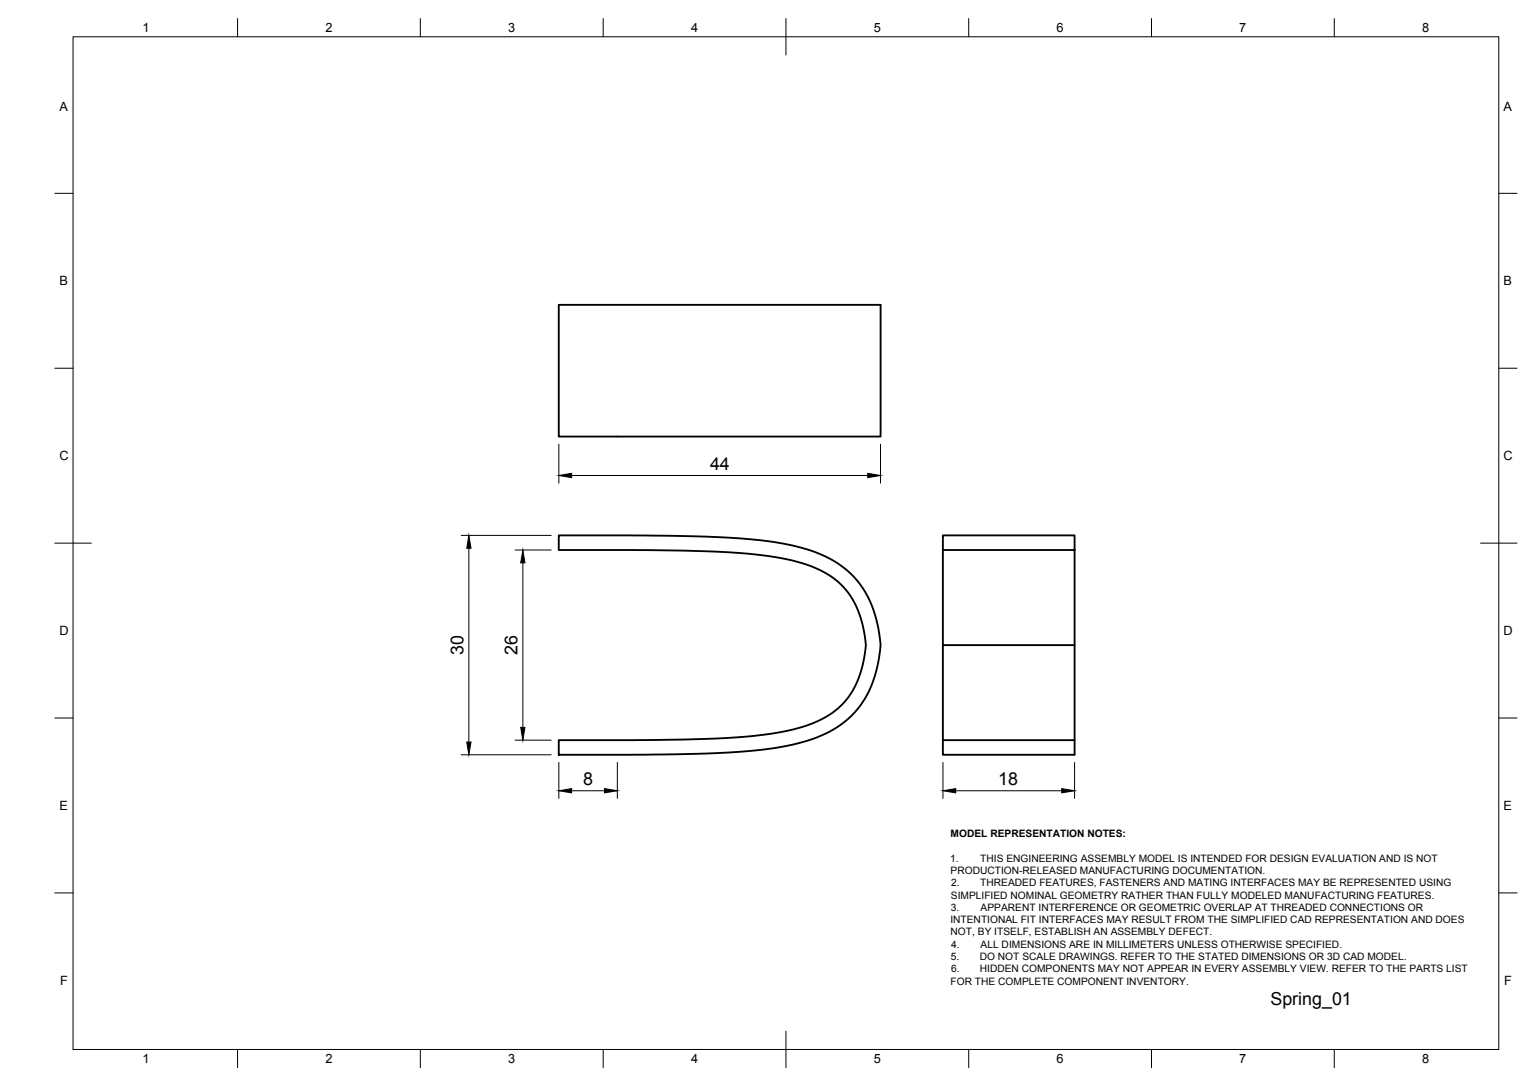
ISO-10303-21;
HEADER;
/* Generated by software containing ST-Developer
 * from STEP Tools, Inc. (www.steptools.com) 
 */

FILE_DESCRIPTION(
/* description */ (''),
/* implementation_level */ '2;1');

FILE_NAME(
/* name */ 'Spring_01.step',
/* time_stamp */ '2026-10-06T13:31:15-07:00',
/* author */ (''),
/* organization */ (''),
/* preprocessor_version */ 'ST-DEVELOPER v20.2',
/* originating_system */ 'Autodesk Translation Framework v15.15.0.0',
/* authorisation */ '');

FILE_SCHEMA (('AUTOMOTIVE_DESIGN { 1 0 10303 214 3 1 1 }'));
ENDSEC;

DATA;
#10=MECHANICAL_DESIGN_GEOMETRIC_PRESENTATION_REPRESENTATION('',(#85),#3154);
#55=B_SPLINE_SURFACE_WITH_KNOTS('',5,1,((#2342,#2343),(#2344,#2345),(#2346,
#2347),(#2348,#2349),(#2350,#2351),(#2352,#2353),(#2354,#2355),(#2356,#2357),
(#2358,#2359),(#2360,#2361),(#2362,#2363),(#2364,#2365),(#2366,#2367),(#2368,
#2369),(#2370,#2371),(#2372,#2373),(#2374,#2375),(#2376,#2377),(#2378,#2379),
(#2380,#2381)),.UNSPECIFIED.,.F.,.F.,.F.,(6,1,1,1,1,1,1,1,1,1,1,1,1,1,1,
6),(2,2),(-1.,-0.933333333333333,-0.866666666666667,-0.8,-0.733333333333333,
-0.666666666666667,-0.6,-0.533333333333333,-0.466666666666667,-0.4,-0.333333333333333,
-0.266666666666667,-0.2,-0.133333333333333,-0.0666666666666667,0.),(0.,
2.16),.UNSPECIFIED.);
#56=B_SPLINE_SURFACE_WITH_KNOTS('',5,1,((#2406,#2407),(#2408,#2409),(#2410,
#2411),(#2412,#2413),(#2414,#2415),(#2416,#2417),(#2418,#2419),(#2420,#2421),
(#2422,#2423),(#2424,#2425),(#2426,#2427),(#2428,#2429),(#2430,#2431),(#2432,
#2433),(#2434,#2435),(#2436,#2437),(#2438,#2439),(#2440,#2441),(#2442,#2443),
(#2444,#2445)),.UNSPECIFIED.,.F.,.F.,.F.,(6,1,1,1,1,1,1,1,1,1,1,1,1,1,1,
6),(2,2),(0.,0.0666666666666667,0.133333333333333,0.2,0.266666666666667,
0.333333333333333,0.4,0.466666666666667,0.533333333333333,0.6,0.666666666666667,
0.733333333333333,0.8,0.866666666666667,0.933333333333333,1.),(0.,2.16),
 .UNSPECIFIED.);
#57=B_SPLINE_SURFACE_WITH_KNOTS('',3,1,((#2480,#2481),(#2482,#2483),(#2484,
#2485),(#2486,#2487),(#2488,#2489),(#2490,#2491),(#2492,#2493),(#2494,#2495),
(#2496,#2497),(#2498,#2499),(#2500,#2501),(#2502,#2503),(#2504,#2505)),
 .UNSPECIFIED.,.F.,.F.,.F.,(4,3,3,3,4),(2,2),(-0.996324238316733,-0.869068416619454,
-0.625,-0.25,0.),(0.,2.16230058202055),.UNSPECIFIED.);
#58=B_SPLINE_SURFACE_WITH_KNOTS('',3,1,((#2518,#2519),(#2520,#2521),(#2522,
#2523),(#2524,#2525),(#2526,#2527),(#2528,#2529),(#2530,#2531),(#2532,#2533),
(#2534,#2535),(#2536,#2537),(#2538,#2539),(#2540,#2541),(#2542,#2543)),
 .UNSPECIFIED.,.F.,.F.,.F.,(4,3,3,3,4),(2,2),(0.,0.25,0.625,0.869068416619454,
0.996324238316631),(0.,2.16230058202055),.UNSPECIFIED.);
#67=SHAPE_REPRESENTATION_RELATIONSHIP('SRR','None',#3195,#76);
#76=ADVANCED_BREP_SHAPE_REPRESENTATION('',(#94),#3151);
#85=STYLED_ITEM('',(#3243),#94);
#94=MANIFOLD_SOLID_BREP('Body1',#1087);
#116=PLANE('',#1249);
#117=PLANE('',#1250);
#118=PLANE('',#1251);
#119=PLANE('',#1252);
#120=PLANE('',#1253);
#121=PLANE('',#1254);
#122=PLANE('',#1255);
#123=PLANE('',#1256);
#206=FACE_OUTER_BOUND('',#270,.T.);
#207=FACE_OUTER_BOUND('',#271,.T.);
#208=FACE_OUTER_BOUND('',#272,.T.);
#209=FACE_OUTER_BOUND('',#273,.T.);
#210=FACE_OUTER_BOUND('',#274,.T.);
#211=FACE_OUTER_BOUND('',#275,.T.);
#212=FACE_OUTER_BOUND('',#276,.T.);
#213=FACE_OUTER_BOUND('',#277,.T.);
#214=FACE_OUTER_BOUND('',#278,.T.);
#215=FACE_OUTER_BOUND('',#279,.T.);
#216=FACE_OUTER_BOUND('',#280,.T.);
#217=FACE_OUTER_BOUND('',#281,.T.);
#270=EDGE_LOOP('',(#868,#869,#870,#871,#872,#873,#874,#875,#876,#877));
#271=EDGE_LOOP('',(#878,#879,#880,#881));
#272=EDGE_LOOP('',(#882,#883,#884,#885));
#273=EDGE_LOOP('',(#886,#887,#888,#889));
#274=EDGE_LOOP('',(#890,#891,#892,#893));
#275=EDGE_LOOP('',(#894,#895,#896,#897));
#276=EDGE_LOOP('',(#898,#899,#900,#901));
#277=EDGE_LOOP('',(#902,#903,#904,#905));
#278=EDGE_LOOP('',(#906,#907,#908,#909));
#279=EDGE_LOOP('',(#910,#911,#912,#913));
#280=EDGE_LOOP('',(#914,#915,#916,#917));
#281=EDGE_LOOP('',(#918,#919,#920,#921,#922,#923,#924,#925,#926,#927));
#333=LINE('',#2268,#399);
#334=LINE('',#2312,#400);
#335=LINE('',#2314,#401);
#336=LINE('',#2316,#402);
#337=LINE('',#2340,#403);
#338=LINE('',#2341,#404);
#339=LINE('',#2383,#405);
#340=LINE('',#2405,#406);
#341=LINE('',#2467,#407);
#342=LINE('',#2470,#408);
#343=LINE('',#2471,#409);
#344=LINE('',#2474,#410);
#345=LINE('',#2475,#411);
#346=LINE('',#2478,#412);
#347=LINE('',#2479,#413);
#348=LINE('',#2517,#414);
#349=LINE('',#2555,#415);
#350=LINE('',#2558,#416);
#351=LINE('',#2559,#417);
#352=LINE('',#2562,#418);
#353=LINE('',#2563,#419);
#354=LINE('',#2565,#420);
#399=VECTOR('',#1439,10.);
#400=VECTOR('',#1440,10.);
#401=VECTOR('',#1441,10.);
#402=VECTOR('',#1442,10.);
#403=VECTOR('',#1443,10.);
#404=VECTOR('',#1444,10.);
#405=VECTOR('',#1445,10.);
#406=VECTOR('',#1446,10.);
#407=VECTOR('',#1447,10.);
#408=VECTOR('',#1450,10.);
#409=VECTOR('',#1451,10.);
#410=VECTOR('',#1454,10.);
#411=VECTOR('',#1455,10.);
#412=VECTOR('',#1458,10.);
#413=VECTOR('',#1459,10.);
#414=VECTOR('',#1460,10.);
#415=VECTOR('',#1461,10.);
#416=VECTOR('',#1464,10.);
#417=VECTOR('',#1465,10.);
#418=VECTOR('',#1468,10.);
#419=VECTOR('',#1469,10.);
#420=VECTOR('',#1472,10.);
#450=B_SPLINE_CURVE_WITH_KNOTS('',5,(#2270,#2271,#2272,#2273,#2274,#2275,
#2276,#2277,#2278,#2279,#2280,#2281,#2282,#2283,#2284,#2285,#2286,#2287,
#2288,#2289),.UNSPECIFIED.,.F.,.F.,(6,1,1,1,1,1,1,1,1,1,1,1,1,1,1,6),(0.,
0.0666666666666667,0.133333333333333,0.2,0.266666666666667,0.333333333333333,
0.4,0.466666666666667,0.533333333333333,0.6,0.666666666666667,0.733333333333333,
0.8,0.866666666666667,0.933333333333333,1.),.UNSPECIFIED.);
#451=B_SPLINE_CURVE_WITH_KNOTS('',5,(#2291,#2292,#2293,#2294,#2295,#2296,
#2297,#2298,#2299,#2300,#2301,#2302,#2303,#2304,#2305,#2306,#2307,#2308,
#2309,#2310),.UNSPECIFIED.,.F.,.F.,(6,1,1,1,1,1,1,1,1,1,1,1,1,1,1,6),(-1.,
-0.933333333333333,-0.866666666666667,-0.8,-0.733333333333333,-0.666666666666667,
-0.6,-0.533333333333333,-0.466666666666667,-0.4,-0.333333333333333,-0.266666666666667,
-0.2,-0.133333333333333,-0.0666666666666667,0.),.UNSPECIFIED.);
#452=B_SPLINE_CURVE_WITH_KNOTS('',3,(#2318,#2319,#2320,#2321,#2322,#2323,
#2324,#2325,#2326,#2327),.UNSPECIFIED.,.F.,.F.,(4,2,2,2,4),(0.,0.249999999999997,
0.624999999999999,0.869068416619453,0.996324238316733),.UNSPECIFIED.);
#453=B_SPLINE_CURVE_WITH_KNOTS('',3,(#2329,#2330,#2331,#2332,#2333,#2334,
#2335,#2336,#2337,#2338),.UNSPECIFIED.,.F.,.F.,(4,2,2,2,4),(-0.996324238316631,
-0.869068416619454,-0.625,-0.25,0.),.UNSPECIFIED.);
#454=B_SPLINE_CURVE_WITH_KNOTS('',5,(#2385,#2386,#2387,#2388,#2389,#2390,
#2391,#2392,#2393,#2394,#2395,#2396,#2397,#2398,#2399,#2400,#2401,#2402,
#2403,#2404),.UNSPECIFIED.,.F.,.F.,(6,1,1,1,1,1,1,1,1,1,1,1,1,1,1,6),(-1.,
-0.933333333333333,-0.866666666666667,-0.8,-0.733333333333333,-0.666666666666667,
-0.6,-0.533333333333333,-0.466666666666667,-0.4,-0.333333333333333,-0.266666666666667,
-0.2,-0.133333333333333,-0.0666666666666667,0.),.UNSPECIFIED.);
#455=B_SPLINE_CURVE_WITH_KNOTS('',5,(#2447,#2448,#2449,#2450,#2451,#2452,
#2453,#2454,#2455,#2456,#2457,#2458,#2459,#2460,#2461,#2462,#2463,#2464,
#2465,#2466),.UNSPECIFIED.,.F.,.F.,(6,1,1,1,1,1,1,1,1,1,1,1,1,1,1,6),(0.,
0.0666666666666667,0.133333333333333,0.2,0.266666666666667,0.333333333333333,
0.4,0.466666666666667,0.533333333333333,0.6,0.666666666666667,0.733333333333333,
0.8,0.866666666666667,0.933333333333333,1.),.UNSPECIFIED.);
#456=B_SPLINE_CURVE_WITH_KNOTS('',3,(#2507,#2508,#2509,#2510,#2511,#2512,
#2513,#2514,#2515,#2516),.UNSPECIFIED.,.F.,.F.,(4,2,2,2,4),(-0.996324238316733,
-0.869068416619454,-0.625,-0.25,0.),.UNSPECIFIED.);
#457=B_SPLINE_CURVE_WITH_KNOTS('',3,(#2545,#2546,#2547,#2548,#2549,#2550,
#2551,#2552,#2553,#2554),.UNSPECIFIED.,.F.,.F.,(4,2,2,2,4),(0.,0.25,0.625,
0.869068416619454,0.996324238316631),.UNSPECIFIED.);
#528=VERTEX_POINT('',#2266);
#529=VERTEX_POINT('',#2267);
#530=VERTEX_POINT('',#2269);
#531=VERTEX_POINT('',#2290);
#532=VERTEX_POINT('',#2311);
#533=VERTEX_POINT('',#2313);
#534=VERTEX_POINT('',#2315);
#535=VERTEX_POINT('',#2317);
#536=VERTEX_POINT('',#2328);
#537=VERTEX_POINT('',#2339);
#538=VERTEX_POINT('',#2382);
#539=VERTEX_POINT('',#2384);
#540=VERTEX_POINT('',#2446);
#541=VERTEX_POINT('',#2469);
#542=VERTEX_POINT('',#2473);
#543=VERTEX_POINT('',#2477);
#544=VERTEX_POINT('',#2506);
#545=VERTEX_POINT('',#2544);
#546=VERTEX_POINT('',#2557);
#547=VERTEX_POINT('',#2561);
#650=EDGE_CURVE('',#528,#529,#333,.T.);
#651=EDGE_CURVE('',#529,#530,#450,.T.);
#652=EDGE_CURVE('',#530,#531,#451,.T.);
#653=EDGE_CURVE('',#531,#532,#334,.T.);
#654=EDGE_CURVE('',#532,#533,#335,.T.);
#655=EDGE_CURVE('',#533,#534,#336,.T.);
#656=EDGE_CURVE('',#534,#535,#452,.T.);
#657=EDGE_CURVE('',#535,#536,#453,.T.);
#658=EDGE_CURVE('',#536,#537,#337,.T.);
#659=EDGE_CURVE('',#537,#528,#338,.T.);
#660=EDGE_CURVE('',#538,#529,#339,.T.);
#661=EDGE_CURVE('',#539,#538,#454,.T.);
#662=EDGE_CURVE('',#530,#539,#340,.T.);
#663=EDGE_CURVE('',#540,#539,#455,.T.);
#664=EDGE_CURVE('',#531,#540,#341,.T.);
#665=EDGE_CURVE('',#541,#540,#342,.T.);
#666=EDGE_CURVE('',#532,#541,#343,.T.);
#667=EDGE_CURVE('',#542,#541,#344,.T.);
#668=EDGE_CURVE('',#533,#542,#345,.T.);
#669=EDGE_CURVE('',#543,#542,#346,.T.);
#670=EDGE_CURVE('',#534,#543,#347,.T.);
#671=EDGE_CURVE('',#544,#543,#456,.T.);
#672=EDGE_CURVE('',#535,#544,#348,.T.);
#673=EDGE_CURVE('',#545,#544,#457,.T.);
#674=EDGE_CURVE('',#536,#545,#349,.T.);
#675=EDGE_CURVE('',#546,#545,#350,.T.);
#676=EDGE_CURVE('',#537,#546,#351,.T.);
#677=EDGE_CURVE('',#547,#546,#352,.T.);
#678=EDGE_CURVE('',#528,#547,#353,.T.);
#679=EDGE_CURVE('',#538,#547,#354,.T.);
#868=ORIENTED_EDGE('',*,*,#650,.T.);
#869=ORIENTED_EDGE('',*,*,#651,.T.);
#870=ORIENTED_EDGE('',*,*,#652,.T.);
#871=ORIENTED_EDGE('',*,*,#653,.T.);
#872=ORIENTED_EDGE('',*,*,#654,.T.);
#873=ORIENTED_EDGE('',*,*,#655,.T.);
#874=ORIENTED_EDGE('',*,*,#656,.T.);
#875=ORIENTED_EDGE('',*,*,#657,.T.);
#876=ORIENTED_EDGE('',*,*,#658,.T.);
#877=ORIENTED_EDGE('',*,*,#659,.T.);
#878=ORIENTED_EDGE('',*,*,#660,.F.);
#879=ORIENTED_EDGE('',*,*,#661,.F.);
#880=ORIENTED_EDGE('',*,*,#662,.F.);
#881=ORIENTED_EDGE('',*,*,#651,.F.);
#882=ORIENTED_EDGE('',*,*,#662,.T.);
#883=ORIENTED_EDGE('',*,*,#663,.F.);
#884=ORIENTED_EDGE('',*,*,#664,.F.);
#885=ORIENTED_EDGE('',*,*,#652,.F.);
#886=ORIENTED_EDGE('',*,*,#664,.T.);
#887=ORIENTED_EDGE('',*,*,#665,.F.);
#888=ORIENTED_EDGE('',*,*,#666,.F.);
#889=ORIENTED_EDGE('',*,*,#653,.F.);
#890=ORIENTED_EDGE('',*,*,#666,.T.);
#891=ORIENTED_EDGE('',*,*,#667,.F.);
#892=ORIENTED_EDGE('',*,*,#668,.F.);
#893=ORIENTED_EDGE('',*,*,#654,.F.);
#894=ORIENTED_EDGE('',*,*,#668,.T.);
#895=ORIENTED_EDGE('',*,*,#669,.F.);
#896=ORIENTED_EDGE('',*,*,#670,.F.);
#897=ORIENTED_EDGE('',*,*,#655,.F.);
#898=ORIENTED_EDGE('',*,*,#670,.T.);
#899=ORIENTED_EDGE('',*,*,#671,.F.);
#900=ORIENTED_EDGE('',*,*,#672,.F.);
#901=ORIENTED_EDGE('',*,*,#656,.F.);
#902=ORIENTED_EDGE('',*,*,#672,.T.);
#903=ORIENTED_EDGE('',*,*,#673,.F.);
#904=ORIENTED_EDGE('',*,*,#674,.F.);
#905=ORIENTED_EDGE('',*,*,#657,.F.);
#906=ORIENTED_EDGE('',*,*,#674,.T.);
#907=ORIENTED_EDGE('',*,*,#675,.F.);
#908=ORIENTED_EDGE('',*,*,#676,.F.);
#909=ORIENTED_EDGE('',*,*,#658,.F.);
#910=ORIENTED_EDGE('',*,*,#676,.T.);
#911=ORIENTED_EDGE('',*,*,#677,.F.);
#912=ORIENTED_EDGE('',*,*,#678,.F.);
#913=ORIENTED_EDGE('',*,*,#659,.F.);
#914=ORIENTED_EDGE('',*,*,#678,.T.);
#915=ORIENTED_EDGE('',*,*,#679,.F.);
#916=ORIENTED_EDGE('',*,*,#660,.T.);
#917=ORIENTED_EDGE('',*,*,#650,.F.);
#918=ORIENTED_EDGE('',*,*,#679,.T.);
#919=ORIENTED_EDGE('',*,*,#677,.T.);
#920=ORIENTED_EDGE('',*,*,#675,.T.);
#921=ORIENTED_EDGE('',*,*,#673,.T.);
#922=ORIENTED_EDGE('',*,*,#671,.T.);
#923=ORIENTED_EDGE('',*,*,#669,.T.);
#924=ORIENTED_EDGE('',*,*,#667,.T.);
#925=ORIENTED_EDGE('',*,*,#665,.T.);
#926=ORIENTED_EDGE('',*,*,#663,.T.);
#927=ORIENTED_EDGE('',*,*,#661,.T.);
#1057=ADVANCED_FACE('',(#206),#116,.F.);
#1058=ADVANCED_FACE('',(#207),#55,.T.);
#1059=ADVANCED_FACE('',(#208),#56,.T.);
#1060=ADVANCED_FACE('',(#209),#117,.T.);
#1061=ADVANCED_FACE('',(#210),#118,.T.);
#1062=ADVANCED_FACE('',(#211),#119,.T.);
#1063=ADVANCED_FACE('',(#212),#57,.T.);
#1064=ADVANCED_FACE('',(#213),#58,.T.);
#1065=ADVANCED_FACE('',(#214),#120,.T.);
#1066=ADVANCED_FACE('',(#215),#121,.T.);
#1067=ADVANCED_FACE('',(#216),#122,.T.);
#1068=ADVANCED_FACE('',(#217),#123,.T.);
#1087=CLOSED_SHELL('',(#1057,#1058,#1059,#1060,#1061,#1062,#1063,#1064,
#1065,#1066,#1067,#1068));
#1248=AXIS2_PLACEMENT_3D('',#2264,#1435,#1436);
#1249=AXIS2_PLACEMENT_3D('',#2265,#1437,#1438);
#1250=AXIS2_PLACEMENT_3D('',#2468,#1448,#1449);
#1251=AXIS2_PLACEMENT_3D('',#2472,#1452,#1453);
#1252=AXIS2_PLACEMENT_3D('',#2476,#1456,#1457);
#1253=AXIS2_PLACEMENT_3D('',#2556,#1462,#1463);
#1254=AXIS2_PLACEMENT_3D('',#2560,#1466,#1467);
#1255=AXIS2_PLACEMENT_3D('',#2564,#1470,#1471);
#1256=AXIS2_PLACEMENT_3D('',#2566,#1473,#1474);
#1435=DIRECTION('axis',(0.,0.,1.));
#1436=DIRECTION('refdir',(1.,0.,0.));
#1437=DIRECTION('center_axis',(0.,1.,0.));
#1438=DIRECTION('ref_axis',(1.,0.,0.));
#1439=DIRECTION('',(0.,0.,-1.));
#1440=DIRECTION('',(0.,0.,1.));
#1441=DIRECTION('',(-1.,0.,0.));
#1442=DIRECTION('',(0.,0.,-1.));
#1443=DIRECTION('',(0.,0.,1.));
#1444=DIRECTION('',(-1.,0.,0.));
#1445=DIRECTION('',(0.,-1.,0.));
#1446=DIRECTION('',(0.,1.,0.));
#1447=DIRECTION('',(0.,1.,0.));
#1448=DIRECTION('center_axis',(1.,0.,0.));
#1449=DIRECTION('ref_axis',(0.,0.,-1.));
#1450=DIRECTION('',(0.,0.,-1.));
#1451=DIRECTION('',(0.,1.,0.));
#1452=DIRECTION('center_axis',(0.,0.,1.));
#1453=DIRECTION('ref_axis',(1.,0.,0.));
#1454=DIRECTION('',(1.,0.,0.));
#1455=DIRECTION('',(0.,1.,0.));
#1456=DIRECTION('center_axis',(-1.,0.,0.));
#1457=DIRECTION('ref_axis',(0.,0.,1.));
#1458=DIRECTION('',(0.,0.,1.));
#1459=DIRECTION('',(0.,1.,0.));
#1460=DIRECTION('',(0.,1.,0.));
#1461=DIRECTION('',(0.,1.,0.));
#1462=DIRECTION('center_axis',(1.,0.,0.));
#1463=DIRECTION('ref_axis',(0.,0.,-1.));
#1464=DIRECTION('',(0.,0.,-1.));
#1465=DIRECTION('',(0.,1.,0.));
#1466=DIRECTION('center_axis',(0.,0.,1.));
#1467=DIRECTION('ref_axis',(1.,0.,0.));
#1468=DIRECTION('',(1.,0.,0.));
#1469=DIRECTION('',(0.,1.,0.));
#1470=DIRECTION('center_axis',(-1.,0.,0.));
#1471=DIRECTION('ref_axis',(0.,0.,1.));
#1472=DIRECTION('',(0.,0.,1.));
#1473=DIRECTION('center_axis',(0.,1.,0.));
#1474=DIRECTION('ref_axis',(1.,0.,0.));
#2264=CARTESIAN_POINT('',(0.,0.,0.));
#2265=CARTESIAN_POINT('Origin',(0.,-9.,162.));
#2266=CARTESIAN_POINT('',(-15.,-9.,184.));
#2267=CARTESIAN_POINT('',(-15.,-9.,176.));
#2268=CARTESIAN_POINT('',(-15.,-9.,184.));
#2269=CARTESIAN_POINT('',(0.,-9.,140.));
#2270=CARTESIAN_POINT('Ctrl Pts',(-15.,-9.,176.));
#2271=CARTESIAN_POINT('Ctrl Pts',(-15.,-9.,175.50441646936));
#2272=CARTESIAN_POINT('Ctrl Pts',(-14.9985513080952,-9.,174.491917916066));
#2273=CARTESIAN_POINT('Ctrl Pts',(-14.9920318646118,-9.,172.909176752281));
#2274=CARTESIAN_POINT('Ctrl Pts',(-14.9745170477256,-9.,170.674187150777));
#2275=CARTESIAN_POINT('Ctrl Pts',(-14.9338349467122,-9.,167.69587590639));
#2276=CARTESIAN_POINT('Ctrl Pts',(-14.8634487703245,-9.,164.57015716772));
#2277=CARTESIAN_POINT('Ctrl Pts',(-14.7422790149997,-9.,161.348120547886));
#2278=CARTESIAN_POINT('Ctrl Pts',(-14.5359735439045,-9.,158.095070696299));
#2279=CARTESIAN_POINT('Ctrl Pts',(-14.1926929497518,-9.,154.892205598351));
#2280=CARTESIAN_POINT('Ctrl Pts',(-13.6496061172615,-9.,151.82914277586));
#2281=CARTESIAN_POINT('Ctrl Pts',(-12.8403951587419,-9.,148.995763819941));
#2282=CARTESIAN_POINT('Ctrl Pts',(-11.7033484644208,-9.,146.473438815185));
#2283=CARTESIAN_POINT('Ctrl Pts',(-10.1890242800701,-9.,144.326851421562));
#2284=CARTESIAN_POINT('Ctrl Pts',(-8.27234033482616,-9.,142.590975648728));
#2285=CARTESIAN_POINT('Ctrl Pts',(-5.94806288019228,-9.,141.276448102944));
#2286=CARTESIAN_POINT('Ctrl Pts',(-3.76616670029465,-9.,140.560219196132));
#2287=CARTESIAN_POINT('Ctrl Pts',(-1.9517913938126,-9.,140.208504145521));
#2288=CARTESIAN_POINT('Ctrl Pts',(-0.663684240665688,-9.,140.055862403662));
#2289=CARTESIAN_POINT('Ctrl Pts',(0.,-9.,140.));
#2290=CARTESIAN_POINT('',(15.,-9.,176.));
#2291=CARTESIAN_POINT('Ctrl Pts',(0.,-9.,140.));
#2292=CARTESIAN_POINT('Ctrl Pts',(0.663684240665688,-9.,140.055862403662));
#2293=CARTESIAN_POINT('Ctrl Pts',(1.9517913938126,-9.,140.208504145521));
#2294=CARTESIAN_POINT('Ctrl Pts',(3.76616670029465,-9.,140.560219196132));
#2295=CARTESIAN_POINT('Ctrl Pts',(5.94806288019228,-9.,141.276448102944));
#2296=CARTESIAN_POINT('Ctrl Pts',(8.27234033482616,-9.,142.590975648728));
#2297=CARTESIAN_POINT('Ctrl Pts',(10.1890242800701,-9.,144.326851421562));
#2298=CARTESIAN_POINT('Ctrl Pts',(11.7033484644208,-9.,146.473438815185));
#2299=CARTESIAN_POINT('Ctrl Pts',(12.8403951587419,-9.,148.995763819941));
#2300=CARTESIAN_POINT('Ctrl Pts',(13.6496061172615,-9.,151.82914277586));
#2301=CARTESIAN_POINT('Ctrl Pts',(14.1926929497518,-9.,154.892205598351));
#2302=CARTESIAN_POINT('Ctrl Pts',(14.5359735439045,-9.,158.095070696299));
#2303=CARTESIAN_POINT('Ctrl Pts',(14.7422790149997,-9.,161.348120547886));
#2304=CARTESIAN_POINT('Ctrl Pts',(14.8634487703245,-9.,164.57015716772));
#2305=CARTESIAN_POINT('Ctrl Pts',(14.9338349467122,-9.,167.69587590639));
#2306=CARTESIAN_POINT('Ctrl Pts',(14.9745170477256,-9.,170.674187150777));
#2307=CARTESIAN_POINT('Ctrl Pts',(14.9920318646118,-9.,172.909176752281));
#2308=CARTESIAN_POINT('Ctrl Pts',(14.9985513080952,-9.,174.491917916066));
#2309=CARTESIAN_POINT('Ctrl Pts',(15.,-9.,175.50441646936));
#2310=CARTESIAN_POINT('Ctrl Pts',(15.,-9.,176.));
#2311=CARTESIAN_POINT('',(15.,-9.,184.));
#2312=CARTESIAN_POINT('',(15.,-9.,184.));
#2313=CARTESIAN_POINT('',(13.,-9.,184.));
#2314=CARTESIAN_POINT('',(-15.,-9.,184.));
#2315=CARTESIAN_POINT('',(13.,-9.,176.));
#2316=CARTESIAN_POINT('',(13.,-9.,184.));
#2317=CARTESIAN_POINT('',(-2.28039809258007E-12,-9.,142.007690234858));
#2318=CARTESIAN_POINT('Ctrl Pts',(13.,-9.,176.));
#2319=CARTESIAN_POINT('Ctrl Pts',(13.,-9.,172.917218954967));
#2320=CARTESIAN_POINT('Ctrl Pts',(12.9804665025967,-9.,169.284971969759));
#2321=CARTESIAN_POINT('Ctrl Pts',(12.7151010160305,-9.,159.547166753218));
#2322=CARTESIAN_POINT('Ctrl Pts',(12.3613339472215,-9.,153.114195242939));
#2323=CARTESIAN_POINT('Ctrl Pts',(9.34288544909169,-9.,146.13723179047));
#2324=CARTESIAN_POINT('Ctrl Pts',(7.62598372131269,-9.,144.320800585332));
#2325=CARTESIAN_POINT('Ctrl Pts',(3.58089918248363,-9.,142.584441583133));
#2326=CARTESIAN_POINT('Ctrl Pts',(1.92777602497513,-9.,142.18420900116));
#2327=CARTESIAN_POINT('Ctrl Pts',(-2.18252499406546E-12,-9.,142.007690234858));
#2328=CARTESIAN_POINT('',(-13.,-9.,176.));
#2329=CARTESIAN_POINT('Ctrl Pts',(-2.28102259303142E-12,-9.,142.007690234858));
#2330=CARTESIAN_POINT('Ctrl Pts',(-1.9277760249776,-9.,142.184209001161));
#2331=CARTESIAN_POINT('Ctrl Pts',(-3.58089918248474,-9.,142.584441583133));
#2332=CARTESIAN_POINT('Ctrl Pts',(-7.62598372131269,-9.,144.320800585332));
#2333=CARTESIAN_POINT('Ctrl Pts',(-9.34288544909169,-9.,146.13723179047));
#2334=CARTESIAN_POINT('Ctrl Pts',(-12.3613339472215,-9.,153.114195242939));
#2335=CARTESIAN_POINT('Ctrl Pts',(-12.7151010160305,-9.,159.547166753218));
#2336=CARTESIAN_POINT('Ctrl Pts',(-12.9804665025967,-9.,169.284971969759));
#2337=CARTESIAN_POINT('Ctrl Pts',(-13.,-9.,172.917218954967));
#2338=CARTESIAN_POINT('Ctrl Pts',(-13.,-9.,176.));
#2339=CARTESIAN_POINT('',(-13.,-9.,184.));
#2340=CARTESIAN_POINT('',(-13.,-9.,184.));
#2341=CARTESIAN_POINT('',(-15.,-9.,184.));
#2342=CARTESIAN_POINT('Ctrl Pts',(0.,-9.,140.));
#2343=CARTESIAN_POINT('Ctrl Pts',(0.,12.6,140.));
#2344=CARTESIAN_POINT('Ctrl Pts',(-0.663684240665688,-9.,140.055862403662));
#2345=CARTESIAN_POINT('Ctrl Pts',(-0.663684240665688,12.6,140.055862403662));
#2346=CARTESIAN_POINT('Ctrl Pts',(-1.9517913938126,-9.,140.208504145521));
#2347=CARTESIAN_POINT('Ctrl Pts',(-1.9517913938126,12.6,140.208504145521));
#2348=CARTESIAN_POINT('Ctrl Pts',(-3.76616670029465,-9.,140.560219196132));
#2349=CARTESIAN_POINT('Ctrl Pts',(-3.76616670029465,12.6,140.560219196132));
#2350=CARTESIAN_POINT('Ctrl Pts',(-5.94806288019228,-9.,141.276448102944));
#2351=CARTESIAN_POINT('Ctrl Pts',(-5.94806288019228,12.6,141.276448102944));
#2352=CARTESIAN_POINT('Ctrl Pts',(-8.27234033482616,-9.,142.590975648728));
#2353=CARTESIAN_POINT('Ctrl Pts',(-8.27234033482616,12.6,142.590975648728));
#2354=CARTESIAN_POINT('Ctrl Pts',(-10.1890242800701,-9.,144.326851421562));
#2355=CARTESIAN_POINT('Ctrl Pts',(-10.1890242800701,12.6,144.326851421562));
#2356=CARTESIAN_POINT('Ctrl Pts',(-11.7033484644208,-9.,146.473438815185));
#2357=CARTESIAN_POINT('Ctrl Pts',(-11.7033484644208,12.6,146.473438815185));
#2358=CARTESIAN_POINT('Ctrl Pts',(-12.8403951587419,-9.,148.995763819941));
#2359=CARTESIAN_POINT('Ctrl Pts',(-12.8403951587419,12.6,148.995763819941));
#2360=CARTESIAN_POINT('Ctrl Pts',(-13.6496061172615,-9.,151.82914277586));
#2361=CARTESIAN_POINT('Ctrl Pts',(-13.6496061172615,12.6,151.82914277586));
#2362=CARTESIAN_POINT('Ctrl Pts',(-14.1926929497518,-9.,154.892205598351));
#2363=CARTESIAN_POINT('Ctrl Pts',(-14.1926929497518,12.6,154.892205598351));
#2364=CARTESIAN_POINT('Ctrl Pts',(-14.5359735439045,-9.,158.095070696299));
#2365=CARTESIAN_POINT('Ctrl Pts',(-14.5359735439045,12.6,158.095070696299));
#2366=CARTESIAN_POINT('Ctrl Pts',(-14.7422790149997,-9.,161.348120547886));
#2367=CARTESIAN_POINT('Ctrl Pts',(-14.7422790149997,12.6,161.348120547886));
#2368=CARTESIAN_POINT('Ctrl Pts',(-14.8634487703245,-9.,164.57015716772));
#2369=CARTESIAN_POINT('Ctrl Pts',(-14.8634487703245,12.6,164.57015716772));
#2370=CARTESIAN_POINT('Ctrl Pts',(-14.9338349467122,-9.,167.69587590639));
#2371=CARTESIAN_POINT('Ctrl Pts',(-14.9338349467122,12.6,167.69587590639));
#2372=CARTESIAN_POINT('Ctrl Pts',(-14.9745170477256,-9.,170.674187150777));
#2373=CARTESIAN_POINT('Ctrl Pts',(-14.9745170477256,12.6,170.674187150777));
#2374=CARTESIAN_POINT('Ctrl Pts',(-14.9920318646118,-9.,172.909176752281));
#2375=CARTESIAN_POINT('Ctrl Pts',(-14.9920318646118,12.6,172.909176752281));
#2376=CARTESIAN_POINT('Ctrl Pts',(-14.9985513080952,-9.,174.491917916066));
#2377=CARTESIAN_POINT('Ctrl Pts',(-14.9985513080952,12.6,174.491917916066));
#2378=CARTESIAN_POINT('Ctrl Pts',(-15.,-9.,175.50441646936));
#2379=CARTESIAN_POINT('Ctrl Pts',(-15.,12.6,175.50441646936));
#2380=CARTESIAN_POINT('Ctrl Pts',(-15.,-9.,176.));
#2381=CARTESIAN_POINT('Ctrl Pts',(-15.,12.6,176.));
#2382=CARTESIAN_POINT('',(-15.,9.,176.));
#2383=CARTESIAN_POINT('',(-15.,0.,176.));
#2384=CARTESIAN_POINT('',(0.,9.,140.));
#2385=CARTESIAN_POINT('Ctrl Pts',(0.,9.,140.));
#2386=CARTESIAN_POINT('Ctrl Pts',(-0.663684240665688,9.,140.055862403662));
#2387=CARTESIAN_POINT('Ctrl Pts',(-1.9517913938126,9.,140.208504145521));
#2388=CARTESIAN_POINT('Ctrl Pts',(-3.76616670029465,9.,140.560219196132));
#2389=CARTESIAN_POINT('Ctrl Pts',(-5.94806288019228,9.,141.276448102944));
#2390=CARTESIAN_POINT('Ctrl Pts',(-8.27234033482616,9.,142.590975648728));
#2391=CARTESIAN_POINT('Ctrl Pts',(-10.1890242800701,9.,144.326851421562));
#2392=CARTESIAN_POINT('Ctrl Pts',(-11.7033484644208,9.,146.473438815185));
#2393=CARTESIAN_POINT('Ctrl Pts',(-12.8403951587419,9.,148.995763819941));
#2394=CARTESIAN_POINT('Ctrl Pts',(-13.6496061172615,9.,151.82914277586));
#2395=CARTESIAN_POINT('Ctrl Pts',(-14.1926929497518,9.,154.892205598351));
#2396=CARTESIAN_POINT('Ctrl Pts',(-14.5359735439045,9.,158.095070696299));
#2397=CARTESIAN_POINT('Ctrl Pts',(-14.7422790149997,9.,161.348120547886));
#2398=CARTESIAN_POINT('Ctrl Pts',(-14.8634487703245,9.,164.57015716772));
#2399=CARTESIAN_POINT('Ctrl Pts',(-14.9338349467122,9.,167.69587590639));
#2400=CARTESIAN_POINT('Ctrl Pts',(-14.9745170477256,9.,170.674187150777));
#2401=CARTESIAN_POINT('Ctrl Pts',(-14.9920318646118,9.,172.909176752281));
#2402=CARTESIAN_POINT('Ctrl Pts',(-14.9985513080952,9.,174.491917916066));
#2403=CARTESIAN_POINT('Ctrl Pts',(-15.,9.,175.50441646936));
#2404=CARTESIAN_POINT('Ctrl Pts',(-15.,9.,176.));
#2405=CARTESIAN_POINT('',(0.,0.,140.));
#2406=CARTESIAN_POINT('Ctrl Pts',(15.,-9.,176.));
#2407=CARTESIAN_POINT('Ctrl Pts',(15.,12.6,176.));
#2408=CARTESIAN_POINT('Ctrl Pts',(15.,-9.,175.50441646936));
#2409=CARTESIAN_POINT('Ctrl Pts',(15.,12.6,175.50441646936));
#2410=CARTESIAN_POINT('Ctrl Pts',(14.9985513080952,-9.,174.491917916066));
#2411=CARTESIAN_POINT('Ctrl Pts',(14.9985513080952,12.6,174.491917916066));
#2412=CARTESIAN_POINT('Ctrl Pts',(14.9920318646118,-9.,172.909176752281));
#2413=CARTESIAN_POINT('Ctrl Pts',(14.9920318646118,12.6,172.909176752281));
#2414=CARTESIAN_POINT('Ctrl Pts',(14.9745170477256,-9.,170.674187150777));
#2415=CARTESIAN_POINT('Ctrl Pts',(14.9745170477256,12.6,170.674187150777));
#2416=CARTESIAN_POINT('Ctrl Pts',(14.9338349467122,-9.,167.69587590639));
#2417=CARTESIAN_POINT('Ctrl Pts',(14.9338349467122,12.6,167.69587590639));
#2418=CARTESIAN_POINT('Ctrl Pts',(14.8634487703245,-9.,164.57015716772));
#2419=CARTESIAN_POINT('Ctrl Pts',(14.8634487703245,12.6,164.57015716772));
#2420=CARTESIAN_POINT('Ctrl Pts',(14.7422790149997,-9.,161.348120547886));
#2421=CARTESIAN_POINT('Ctrl Pts',(14.7422790149997,12.6,161.348120547886));
#2422=CARTESIAN_POINT('Ctrl Pts',(14.5359735439045,-9.,158.095070696299));
#2423=CARTESIAN_POINT('Ctrl Pts',(14.5359735439045,12.6,158.095070696299));
#2424=CARTESIAN_POINT('Ctrl Pts',(14.1926929497518,-9.,154.892205598351));
#2425=CARTESIAN_POINT('Ctrl Pts',(14.1926929497518,12.6,154.892205598351));
#2426=CARTESIAN_POINT('Ctrl Pts',(13.6496061172615,-9.,151.82914277586));
#2427=CARTESIAN_POINT('Ctrl Pts',(13.6496061172615,12.6,151.82914277586));
#2428=CARTESIAN_POINT('Ctrl Pts',(12.8403951587419,-9.,148.995763819941));
#2429=CARTESIAN_POINT('Ctrl Pts',(12.8403951587419,12.6,148.995763819941));
#2430=CARTESIAN_POINT('Ctrl Pts',(11.7033484644208,-9.,146.473438815185));
#2431=CARTESIAN_POINT('Ctrl Pts',(11.7033484644208,12.6,146.473438815185));
#2432=CARTESIAN_POINT('Ctrl Pts',(10.1890242800701,-9.,144.326851421562));
#2433=CARTESIAN_POINT('Ctrl Pts',(10.1890242800701,12.6,144.326851421562));
#2434=CARTESIAN_POINT('Ctrl Pts',(8.27234033482616,-9.,142.590975648728));
#2435=CARTESIAN_POINT('Ctrl Pts',(8.27234033482616,12.6,142.590975648728));
#2436=CARTESIAN_POINT('Ctrl Pts',(5.94806288019228,-9.,141.276448102944));
#2437=CARTESIAN_POINT('Ctrl Pts',(5.94806288019228,12.6,141.276448102944));
#2438=CARTESIAN_POINT('Ctrl Pts',(3.76616670029465,-9.,140.560219196132));
#2439=CARTESIAN_POINT('Ctrl Pts',(3.76616670029465,12.6,140.560219196132));
#2440=CARTESIAN_POINT('Ctrl Pts',(1.9517913938126,-9.,140.208504145521));
#2441=CARTESIAN_POINT('Ctrl Pts',(1.9517913938126,12.6,140.208504145521));
#2442=CARTESIAN_POINT('Ctrl Pts',(0.663684240665688,-9.,140.055862403662));
#2443=CARTESIAN_POINT('Ctrl Pts',(0.663684240665688,12.6,140.055862403662));
#2444=CARTESIAN_POINT('Ctrl Pts',(0.,-9.,140.));
#2445=CARTESIAN_POINT('Ctrl Pts',(0.,12.6,140.));
#2446=CARTESIAN_POINT('',(15.,9.,176.));
#2447=CARTESIAN_POINT('Ctrl Pts',(15.,9.,176.));
#2448=CARTESIAN_POINT('Ctrl Pts',(15.,9.,175.50441646936));
#2449=CARTESIAN_POINT('Ctrl Pts',(14.9985513080952,9.,174.491917916066));
#2450=CARTESIAN_POINT('Ctrl Pts',(14.9920318646118,9.,172.909176752281));
#2451=CARTESIAN_POINT('Ctrl Pts',(14.9745170477256,9.,170.674187150777));
#2452=CARTESIAN_POINT('Ctrl Pts',(14.9338349467122,9.,167.69587590639));
#2453=CARTESIAN_POINT('Ctrl Pts',(14.8634487703245,9.,164.57015716772));
#2454=CARTESIAN_POINT('Ctrl Pts',(14.7422790149997,9.,161.348120547886));
#2455=CARTESIAN_POINT('Ctrl Pts',(14.5359735439045,9.,158.095070696299));
#2456=CARTESIAN_POINT('Ctrl Pts',(14.1926929497518,9.,154.892205598351));
#2457=CARTESIAN_POINT('Ctrl Pts',(13.6496061172615,9.,151.82914277586));
#2458=CARTESIAN_POINT('Ctrl Pts',(12.8403951587419,9.,148.995763819941));
#2459=CARTESIAN_POINT('Ctrl Pts',(11.7033484644208,9.,146.473438815185));
#2460=CARTESIAN_POINT('Ctrl Pts',(10.1890242800701,9.,144.326851421562));
#2461=CARTESIAN_POINT('Ctrl Pts',(8.27234033482616,9.,142.590975648728));
#2462=CARTESIAN_POINT('Ctrl Pts',(5.94806288019228,9.,141.276448102944));
#2463=CARTESIAN_POINT('Ctrl Pts',(3.76616670029465,9.,140.560219196132));
#2464=CARTESIAN_POINT('Ctrl Pts',(1.9517913938126,9.,140.208504145521));
#2465=CARTESIAN_POINT('Ctrl Pts',(0.663684240665688,9.,140.055862403662));
#2466=CARTESIAN_POINT('Ctrl Pts',(0.,9.,140.));
#2467=CARTESIAN_POINT('',(15.,0.,176.));
#2468=CARTESIAN_POINT('Origin',(15.,0.,184.));
#2469=CARTESIAN_POINT('',(15.,9.,184.));
#2470=CARTESIAN_POINT('',(15.,9.,184.));
#2471=CARTESIAN_POINT('',(15.,0.,184.));
#2472=CARTESIAN_POINT('Origin',(13.,0.,184.));
#2473=CARTESIAN_POINT('',(13.,9.,184.));
#2474=CARTESIAN_POINT('',(-15.,9.,184.));
#2475=CARTESIAN_POINT('',(13.,0.,184.));
#2476=CARTESIAN_POINT('Origin',(13.,0.,176.));
#2477=CARTESIAN_POINT('',(13.,9.,176.));
#2478=CARTESIAN_POINT('',(13.,9.,184.));
#2479=CARTESIAN_POINT('',(13.,0.,176.));
#2480=CARTESIAN_POINT('Ctrl Pts',(-2.18252499406546E-12,-9.01917151683795,
142.007690234858));
#2481=CARTESIAN_POINT('Ctrl Pts',(-2.18252499406546E-12,12.6038343033676,
142.007690234858));
#2482=CARTESIAN_POINT('Ctrl Pts',(1.92777602497513,-9.01917151683795,142.18420900116));
#2483=CARTESIAN_POINT('Ctrl Pts',(1.92777602497513,12.6038343033676,142.18420900116));
#2484=CARTESIAN_POINT('Ctrl Pts',(3.58089918248363,-9.01917151683795,142.584441583133));
#2485=CARTESIAN_POINT('Ctrl Pts',(3.58089918248363,12.6038343033676,142.584441583133));
#2486=CARTESIAN_POINT('Ctrl Pts',(4.96718239188881,-9.01917151683795,143.179505866003));
#2487=CARTESIAN_POINT('Ctrl Pts',(4.96718239188881,12.6038343033676,143.179505866003));
#2488=CARTESIAN_POINT('Ctrl Pts',(7.62598372131269,-9.01917151683795,144.320800585332));
#2489=CARTESIAN_POINT('Ctrl Pts',(7.62598372131269,12.6038343033676,144.320800585332));
#2490=CARTESIAN_POINT('Ctrl Pts',(9.34288544909169,-9.01917151683795,146.13723179047));
#2491=CARTESIAN_POINT('Ctrl Pts',(9.34288544909169,12.6038343033676,146.13723179047));
#2492=CARTESIAN_POINT('Ctrl Pts',(10.5329121501934,-9.01917151683795,148.887907445925));
#2493=CARTESIAN_POINT('Ctrl Pts',(10.5329121501934,12.6038343033676,148.887907445925));
#2494=CARTESIAN_POINT('Ctrl Pts',(12.3613339472215,-9.01917151683795,153.114195242939));
#2495=CARTESIAN_POINT('Ctrl Pts',(12.3613339472215,12.6038343033676,153.114195242939));
#2496=CARTESIAN_POINT('Ctrl Pts',(12.7151010160305,-9.01917151683795,159.547166753218));
#2497=CARTESIAN_POINT('Ctrl Pts',(12.7151010160305,12.6038343033676,159.547166753218));
#2498=CARTESIAN_POINT('Ctrl Pts',(12.8743203079702,-9.01917151683795,165.389849883143));
#2499=CARTESIAN_POINT('Ctrl Pts',(12.8743203079702,12.6038343033676,165.389849883143));
#2500=CARTESIAN_POINT('Ctrl Pts',(12.9804665025967,-9.01917151683795,169.284971969759));
#2501=CARTESIAN_POINT('Ctrl Pts',(12.9804665025967,12.6038343033676,169.284971969759));
#2502=CARTESIAN_POINT('Ctrl Pts',(13.,-9.01917151683795,172.917218954967));
#2503=CARTESIAN_POINT('Ctrl Pts',(13.,12.6038343033676,172.917218954967));
#2504=CARTESIAN_POINT('Ctrl Pts',(13.,-9.01917151683795,176.));
#2505=CARTESIAN_POINT('Ctrl Pts',(13.,12.6038343033676,176.));
#2506=CARTESIAN_POINT('',(-2.28039809258007E-12,9.,142.007690234858));
#2507=CARTESIAN_POINT('Ctrl Pts',(-2.18252499406546E-12,9.,142.007690234858));
#2508=CARTESIAN_POINT('Ctrl Pts',(1.92777602497513,9.,142.18420900116));
#2509=CARTESIAN_POINT('Ctrl Pts',(3.58089918248363,9.,142.584441583133));
#2510=CARTESIAN_POINT('Ctrl Pts',(7.62598372131269,9.,144.320800585332));
#2511=CARTESIAN_POINT('Ctrl Pts',(9.34288544909169,9.,146.13723179047));
#2512=CARTESIAN_POINT('Ctrl Pts',(12.3613339472215,9.,153.114195242939));
#2513=CARTESIAN_POINT('Ctrl Pts',(12.7151010160305,9.,159.547166753218));
#2514=CARTESIAN_POINT('Ctrl Pts',(12.9804665025967,9.,169.284971969759));
#2515=CARTESIAN_POINT('Ctrl Pts',(13.,9.,172.917218954967));
#2516=CARTESIAN_POINT('Ctrl Pts',(13.,9.,176.));
#2517=CARTESIAN_POINT('',(-2.28102259303142E-12,0.,142.007690234858));
#2518=CARTESIAN_POINT('Ctrl Pts',(-13.,-9.01917151683795,176.));
#2519=CARTESIAN_POINT('Ctrl Pts',(-13.,12.6038343033676,176.));
#2520=CARTESIAN_POINT('Ctrl Pts',(-13.,-9.01917151683795,172.917218954967));
#2521=CARTESIAN_POINT('Ctrl Pts',(-13.,12.6038343033676,172.917218954967));
#2522=CARTESIAN_POINT('Ctrl Pts',(-12.9804665025967,-9.01917151683795,169.284971969759));
#2523=CARTESIAN_POINT('Ctrl Pts',(-12.9804665025967,12.6038343033676,169.284971969759));
#2524=CARTESIAN_POINT('Ctrl Pts',(-12.8743203079702,-9.01917151683795,165.389849883143));
#2525=CARTESIAN_POINT('Ctrl Pts',(-12.8743203079702,12.6038343033676,165.389849883143));
#2526=CARTESIAN_POINT('Ctrl Pts',(-12.7151010160305,-9.01917151683795,159.547166753218));
#2527=CARTESIAN_POINT('Ctrl Pts',(-12.7151010160305,12.6038343033676,159.547166753218));
#2528=CARTESIAN_POINT('Ctrl Pts',(-12.3613339472215,-9.01917151683795,153.114195242939));
#2529=CARTESIAN_POINT('Ctrl Pts',(-12.3613339472215,12.6038343033676,153.114195242939));
#2530=CARTESIAN_POINT('Ctrl Pts',(-10.5329121501934,-9.01917151683795,148.887907445925));
#2531=CARTESIAN_POINT('Ctrl Pts',(-10.5329121501934,12.6038343033676,148.887907445925));
#2532=CARTESIAN_POINT('Ctrl Pts',(-9.34288544909169,-9.01917151683795,146.13723179047));
#2533=CARTESIAN_POINT('Ctrl Pts',(-9.34288544909169,12.6038343033676,146.13723179047));
#2534=CARTESIAN_POINT('Ctrl Pts',(-7.62598372131269,-9.01917151683795,144.320800585332));
#2535=CARTESIAN_POINT('Ctrl Pts',(-7.62598372131269,12.6038343033676,144.320800585332));
#2536=CARTESIAN_POINT('Ctrl Pts',(-4.96718239188881,-9.01917151683795,143.179505866003));
#2537=CARTESIAN_POINT('Ctrl Pts',(-4.96718239188881,12.6038343033676,143.179505866003));
#2538=CARTESIAN_POINT('Ctrl Pts',(-3.58089918248474,-9.01917151683795,142.584441583133));
#2539=CARTESIAN_POINT('Ctrl Pts',(-3.58089918248474,12.6038343033676,142.584441583133));
#2540=CARTESIAN_POINT('Ctrl Pts',(-1.9277760249776,-9.01917151683795,142.184209001161));
#2541=CARTESIAN_POINT('Ctrl Pts',(-1.9277760249776,12.6038343033676,142.184209001161));
#2542=CARTESIAN_POINT('Ctrl Pts',(-2.28102259303142E-12,-9.01917151683795,
142.007690234858));
#2543=CARTESIAN_POINT('Ctrl Pts',(-2.28102259303142E-12,12.6038343033676,
142.007690234858));
#2544=CARTESIAN_POINT('',(-13.,9.,176.));
#2545=CARTESIAN_POINT('Ctrl Pts',(-13.,9.,176.));
#2546=CARTESIAN_POINT('Ctrl Pts',(-13.,9.,172.917218954967));
#2547=CARTESIAN_POINT('Ctrl Pts',(-12.9804665025967,9.,169.284971969759));
#2548=CARTESIAN_POINT('Ctrl Pts',(-12.7151010160305,9.,159.547166753218));
#2549=CARTESIAN_POINT('Ctrl Pts',(-12.3613339472215,9.,153.114195242939));
#2550=CARTESIAN_POINT('Ctrl Pts',(-9.34288544909169,9.,146.13723179047));
#2551=CARTESIAN_POINT('Ctrl Pts',(-7.62598372131269,9.,144.320800585332));
#2552=CARTESIAN_POINT('Ctrl Pts',(-3.58089918248474,9.,142.584441583133));
#2553=CARTESIAN_POINT('Ctrl Pts',(-1.9277760249776,9.,142.184209001161));
#2554=CARTESIAN_POINT('Ctrl Pts',(-2.28102259303142E-12,9.,142.007690234858));
#2555=CARTESIAN_POINT('',(-13.,0.,176.));
#2556=CARTESIAN_POINT('Origin',(-13.,0.,184.));
#2557=CARTESIAN_POINT('',(-13.,9.,184.));
#2558=CARTESIAN_POINT('',(-13.,9.,184.));
#2559=CARTESIAN_POINT('',(-13.,0.,184.));
#2560=CARTESIAN_POINT('Origin',(-15.,0.,184.));
#2561=CARTESIAN_POINT('',(-15.,9.,184.));
#2562=CARTESIAN_POINT('',(-15.,9.,184.));
#2563=CARTESIAN_POINT('',(-15.,0.,184.));
#2564=CARTESIAN_POINT('Origin',(-15.,0.,176.));
#2565=CARTESIAN_POINT('',(-15.,9.,184.));
#2566=CARTESIAN_POINT('Origin',(0.,9.,162.));
#3140=UNCERTAINTY_MEASURE_WITH_UNIT(LENGTH_MEASURE(0.01),#3155,
'DISTANCE_ACCURACY_VALUE',
'Maximum model space distance between geometric entities at asserted c
onnectivities');
#3143=UNCERTAINTY_MEASURE_WITH_UNIT(LENGTH_MEASURE(0.01),#3155,
'DISTANCE_ACCURACY_VALUE',
'Maximum model space distance between geometric entities at asserted c
onnectivities');
#3151=(
GEOMETRIC_REPRESENTATION_CONTEXT(3)
GLOBAL_UNCERTAINTY_ASSIGNED_CONTEXT((#3140))
GLOBAL_UNIT_ASSIGNED_CONTEXT((#3155,#3157,#3158))
REPRESENTATION_CONTEXT('','3D')
);
#3154=(
GEOMETRIC_REPRESENTATION_CONTEXT(3)
GLOBAL_UNCERTAINTY_ASSIGNED_CONTEXT((#3143))
GLOBAL_UNIT_ASSIGNED_CONTEXT((#3155,#3157,#3158))
REPRESENTATION_CONTEXT('','3D')
);
#3155=(
LENGTH_UNIT()
NAMED_UNIT(*)
SI_UNIT(.MILLI.,.METRE.)
);
#3157=(
NAMED_UNIT(*)
PLANE_ANGLE_UNIT()
SI_UNIT($,.RADIAN.)
);
#3158=(
NAMED_UNIT(*)
SI_UNIT($,.STERADIAN.)
SOLID_ANGLE_UNIT()
);
#3166=SHAPE_DEFINITION_REPRESENTATION(#3176,#3195);
#3176=PRODUCT_DEFINITION_SHAPE('',$,#3206);
#3195=SHAPE_REPRESENTATION('',(#1248),#3151);
#3198=PRODUCT_DEFINITION_CONTEXT('part definition',#3230,'design');
#3206=PRODUCT_DEFINITION('Spring_01','Spring_01',#3216,#3198);
#3216=PRODUCT_DEFINITION_FORMATION('',$,#3239);
#3230=APPLICATION_CONTEXT(
'Core Data for Automotive Mechanical Design Process');
#3231=PRODUCT_CONTEXT('part definition',#3230,'mechanical');
#3239=PRODUCT('Spring_01','Spring_01',$,(#3231));
#3243=PRESENTATION_STYLE_ASSIGNMENT((#3245));
#3245=SURFACE_STYLE_USAGE(.BOTH.,#3247);
#3247=SURFACE_SIDE_STYLE('',(#3249));
#3249=SURFACE_STYLE_FILL_AREA(#3251);
#3251=FILL_AREA_STYLE('Opaque(160,160,160)',(#3253));
#3253=FILL_AREA_STYLE_COLOUR('Opaque(160,160,160)',#3255);
#3255=COLOUR_RGB('Opaque(160,160,160)', 0.09019608, 0.27058824, 0.51372549);
ENDSEC;
END-ISO-10303-21;
